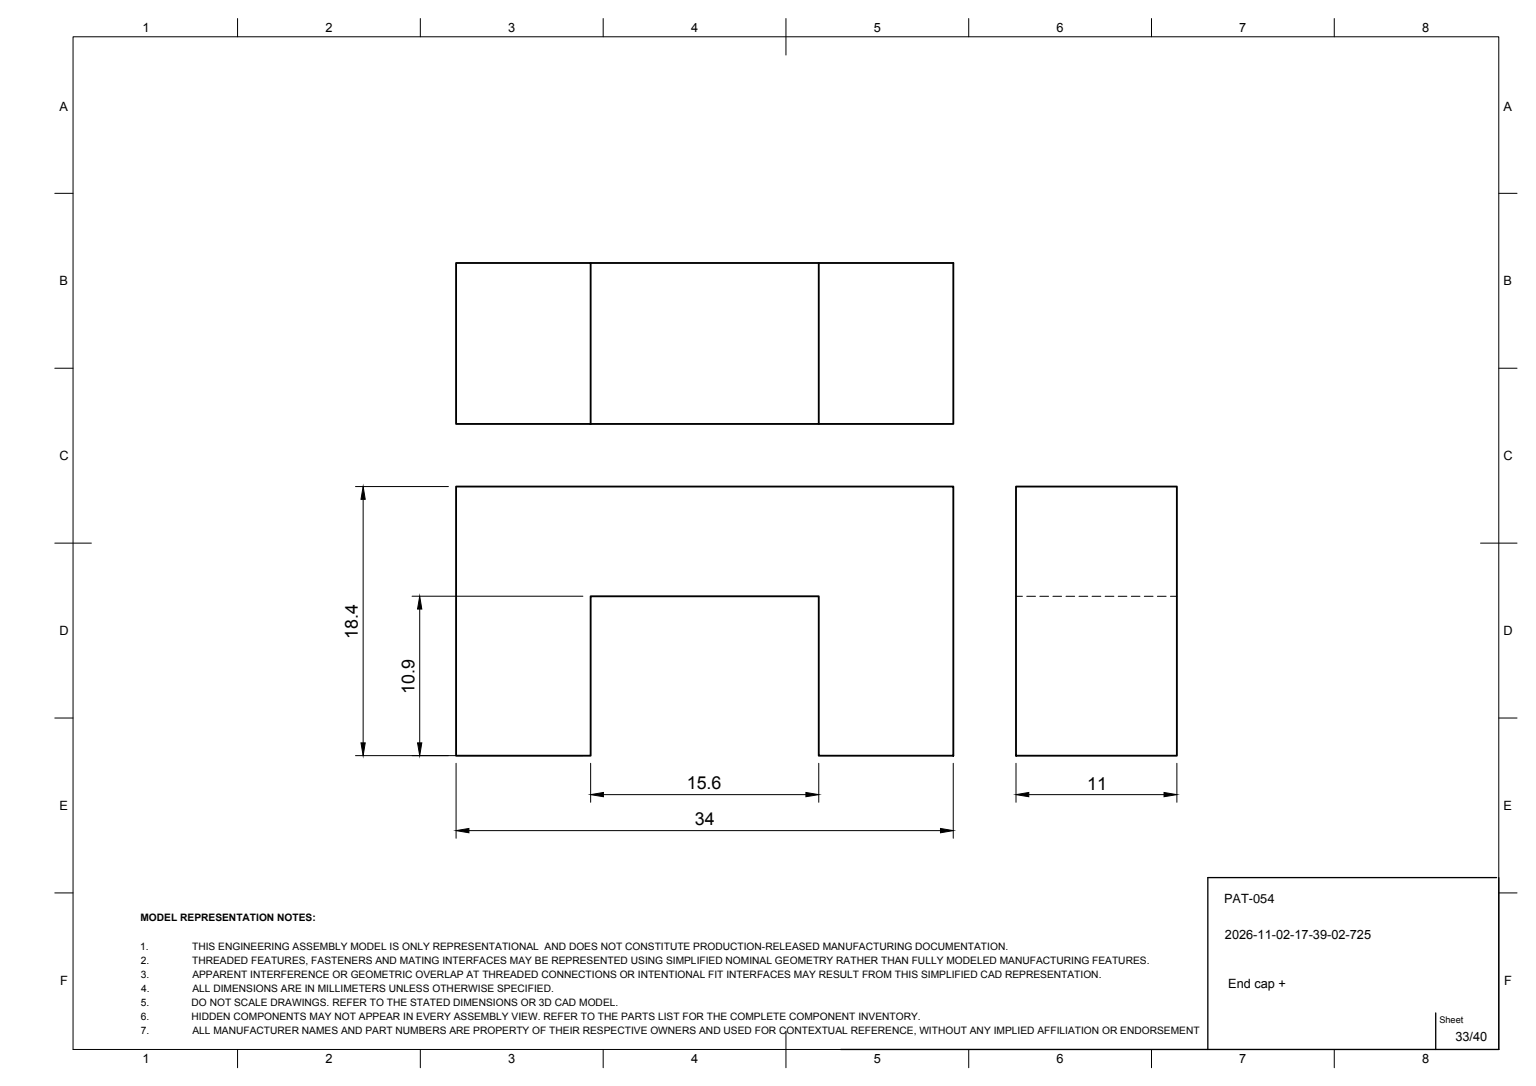
ISO-10303-21;
HEADER;
/* Generated by software containing ST-Developer
 * from STEP Tools, Inc. (www.steptools.com) 
 */

FILE_DESCRIPTION(
/* description */ ('PAT-054'),
/* implementation_level */ '2;1');

FILE_NAME(
/* name */ 'End cap +.step',
/* time_stamp */ '2026-10-29T16:38:13-07:00',
/* author */ (''),
/* organization */ (''),
/* preprocessor_version */ 'ST-DEVELOPER v20.2',
/* originating_system */ 'Autodesk Translation Framework v15.17.0.0',
/* authorisation */ '');

FILE_SCHEMA (('AUTOMOTIVE_DESIGN { 1 0 10303 214 3 1 1 }'));
ENDSEC;

DATA;
#10=MECHANICAL_DESIGN_GEOMETRIC_PRESENTATION_REPRESENTATION('',(#941),#33981);
#838=SHAPE_REPRESENTATION_RELATIONSHIP('SRR','None',#34215,#882);
#882=ADVANCED_BREP_SHAPE_REPRESENTATION('',(#999),#33963);
#941=STYLED_ITEM('',(#34510),#999);
#999=MANIFOLD_SOLID_BREP('Body1',#13053);
#1455=PLANE('',#14365);
#1456=PLANE('',#14366);
#1457=PLANE('',#14367);
#1458=PLANE('',#14368);
#1459=PLANE('',#14369);
#1460=PLANE('',#14370);
#1461=PLANE('',#14371);
#1462=PLANE('',#14372);
#1463=PLANE('',#14373);
#1464=PLANE('',#14374);
#1972=FACE_OUTER_BOUND('',#2872,.T.);
#1973=FACE_OUTER_BOUND('',#2873,.T.);
#1974=FACE_OUTER_BOUND('',#2874,.T.);
#1975=FACE_OUTER_BOUND('',#2875,.T.);
#1976=FACE_OUTER_BOUND('',#2876,.T.);
#1977=FACE_OUTER_BOUND('',#2877,.T.);
#1978=FACE_OUTER_BOUND('',#2878,.T.);
#1979=FACE_OUTER_BOUND('',#2879,.T.);
#1980=FACE_OUTER_BOUND('',#2880,.T.);
#1981=FACE_OUTER_BOUND('',#2881,.T.);
#2872=EDGE_LOOP('',(#10373,#10374,#10375,#10376));
#2873=EDGE_LOOP('',(#10377,#10378,#10379,#10380));
#2874=EDGE_LOOP('',(#10381,#10382,#10383,#10384));
#2875=EDGE_LOOP('',(#10385,#10386,#10387,#10388));
#2876=EDGE_LOOP('',(#10389,#10390,#10391,#10392));
#2877=EDGE_LOOP('',(#10393,#10394,#10395,#10396));
#2878=EDGE_LOOP('',(#10397,#10398,#10399,#10400));
#2879=EDGE_LOOP('',(#10401,#10402,#10403,#10404));
#2880=EDGE_LOOP('',(#10405,#10406,#10407,#10408,#10409,#10410,#10411,#10412));
#2881=EDGE_LOOP('',(#10413,#10414,#10415,#10416,#10417,#10418,#10419,#10420));
#3782=LINE('',#21148,#4716);
#3783=LINE('',#21150,#4717);
#3784=LINE('',#21152,#4718);
#3785=LINE('',#21153,#4719);
#3786=LINE('',#21156,#4720);
#3787=LINE('',#21158,#4721);
#3788=LINE('',#21159,#4722);
#3789=LINE('',#21162,#4723);
#3790=LINE('',#21164,#4724);
#3791=LINE('',#21165,#4725);
#3792=LINE('',#21168,#4726);
#3793=LINE('',#21170,#4727);
#3794=LINE('',#21171,#4728);
#3795=LINE('',#21174,#4729);
#3796=LINE('',#21176,#4730);
#3797=LINE('',#21177,#4731);
#3798=LINE('',#21180,#4732);
#3799=LINE('',#21182,#4733);
#3800=LINE('',#21183,#4734);
#3801=LINE('',#21186,#4735);
#3802=LINE('',#21188,#4736);
#3803=LINE('',#21189,#4737);
#3804=LINE('',#21191,#4738);
#3805=LINE('',#21192,#4739);
#4716=VECTOR('',#17049,1.);
#4717=VECTOR('',#17050,1.);
#4718=VECTOR('',#17051,1.);
#4719=VECTOR('',#17052,1.);
#4720=VECTOR('',#17055,1.);
#4721=VECTOR('',#17056,1.);
#4722=VECTOR('',#17057,1.);
#4723=VECTOR('',#17060,1.);
#4724=VECTOR('',#17061,1.);
#4725=VECTOR('',#17062,1.);
#4726=VECTOR('',#17065,1.);
#4727=VECTOR('',#17066,1.);
#4728=VECTOR('',#17067,1.);
#4729=VECTOR('',#17070,1.);
#4730=VECTOR('',#17071,1.);
#4731=VECTOR('',#17072,1.);
#4732=VECTOR('',#17075,1.);
#4733=VECTOR('',#17076,1.);
#4734=VECTOR('',#17077,1.);
#4735=VECTOR('',#17080,1.);
#4736=VECTOR('',#17081,1.);
#4737=VECTOR('',#17082,1.);
#4738=VECTOR('',#17085,1.);
#4739=VECTOR('',#17086,1.);
#6214=VERTEX_POINT('',#21146);
#6215=VERTEX_POINT('',#21147);
#6216=VERTEX_POINT('',#21149);
#6217=VERTEX_POINT('',#21151);
#6218=VERTEX_POINT('',#21155);
#6219=VERTEX_POINT('',#21157);
#6220=VERTEX_POINT('',#21161);
#6221=VERTEX_POINT('',#21163);
#6222=VERTEX_POINT('',#21167);
#6223=VERTEX_POINT('',#21169);
#6224=VERTEX_POINT('',#21173);
#6225=VERTEX_POINT('',#21175);
#6226=VERTEX_POINT('',#21179);
#6227=VERTEX_POINT('',#21181);
#6228=VERTEX_POINT('',#21185);
#6229=VERTEX_POINT('',#21187);
#7686=EDGE_CURVE('',#6214,#6215,#3782,.T.);
#7687=EDGE_CURVE('',#6215,#6216,#3783,.T.);
#7688=EDGE_CURVE('',#6217,#6216,#3784,.T.);
#7689=EDGE_CURVE('',#6214,#6217,#3785,.T.);
#7690=EDGE_CURVE('',#6218,#6214,#3786,.T.);
#7691=EDGE_CURVE('',#6219,#6217,#3787,.T.);
#7692=EDGE_CURVE('',#6218,#6219,#3788,.T.);
#7693=EDGE_CURVE('',#6220,#6218,#3789,.T.);
#7694=EDGE_CURVE('',#6221,#6219,#3790,.T.);
#7695=EDGE_CURVE('',#6220,#6221,#3791,.T.);
#7696=EDGE_CURVE('',#6222,#6220,#3792,.T.);
#7697=EDGE_CURVE('',#6223,#6221,#3793,.T.);
#7698=EDGE_CURVE('',#6222,#6223,#3794,.T.);
#7699=EDGE_CURVE('',#6224,#6222,#3795,.T.);
#7700=EDGE_CURVE('',#6225,#6223,#3796,.T.);
#7701=EDGE_CURVE('',#6224,#6225,#3797,.T.);
#7702=EDGE_CURVE('',#6226,#6224,#3798,.T.);
#7703=EDGE_CURVE('',#6227,#6225,#3799,.T.);
#7704=EDGE_CURVE('',#6226,#6227,#3800,.T.);
#7705=EDGE_CURVE('',#6228,#6226,#3801,.T.);
#7706=EDGE_CURVE('',#6229,#6227,#3802,.T.);
#7707=EDGE_CURVE('',#6228,#6229,#3803,.T.);
#7708=EDGE_CURVE('',#6215,#6228,#3804,.T.);
#7709=EDGE_CURVE('',#6216,#6229,#3805,.T.);
#10373=ORIENTED_EDGE('',*,*,#7686,.T.);
#10374=ORIENTED_EDGE('',*,*,#7687,.T.);
#10375=ORIENTED_EDGE('',*,*,#7688,.F.);
#10376=ORIENTED_EDGE('',*,*,#7689,.F.);
#10377=ORIENTED_EDGE('',*,*,#7690,.T.);
#10378=ORIENTED_EDGE('',*,*,#7689,.T.);
#10379=ORIENTED_EDGE('',*,*,#7691,.F.);
#10380=ORIENTED_EDGE('',*,*,#7692,.F.);
#10381=ORIENTED_EDGE('',*,*,#7693,.T.);
#10382=ORIENTED_EDGE('',*,*,#7692,.T.);
#10383=ORIENTED_EDGE('',*,*,#7694,.F.);
#10384=ORIENTED_EDGE('',*,*,#7695,.F.);
#10385=ORIENTED_EDGE('',*,*,#7696,.T.);
#10386=ORIENTED_EDGE('',*,*,#7695,.T.);
#10387=ORIENTED_EDGE('',*,*,#7697,.F.);
#10388=ORIENTED_EDGE('',*,*,#7698,.F.);
#10389=ORIENTED_EDGE('',*,*,#7699,.T.);
#10390=ORIENTED_EDGE('',*,*,#7698,.T.);
#10391=ORIENTED_EDGE('',*,*,#7700,.F.);
#10392=ORIENTED_EDGE('',*,*,#7701,.F.);
#10393=ORIENTED_EDGE('',*,*,#7702,.T.);
#10394=ORIENTED_EDGE('',*,*,#7701,.T.);
#10395=ORIENTED_EDGE('',*,*,#7703,.F.);
#10396=ORIENTED_EDGE('',*,*,#7704,.F.);
#10397=ORIENTED_EDGE('',*,*,#7705,.T.);
#10398=ORIENTED_EDGE('',*,*,#7704,.T.);
#10399=ORIENTED_EDGE('',*,*,#7706,.F.);
#10400=ORIENTED_EDGE('',*,*,#7707,.F.);
#10401=ORIENTED_EDGE('',*,*,#7708,.T.);
#10402=ORIENTED_EDGE('',*,*,#7707,.T.);
#10403=ORIENTED_EDGE('',*,*,#7709,.F.);
#10404=ORIENTED_EDGE('',*,*,#7687,.F.);
#10405=ORIENTED_EDGE('',*,*,#7709,.T.);
#10406=ORIENTED_EDGE('',*,*,#7706,.T.);
#10407=ORIENTED_EDGE('',*,*,#7703,.T.);
#10408=ORIENTED_EDGE('',*,*,#7700,.T.);
#10409=ORIENTED_EDGE('',*,*,#7697,.T.);
#10410=ORIENTED_EDGE('',*,*,#7694,.T.);
#10411=ORIENTED_EDGE('',*,*,#7691,.T.);
#10412=ORIENTED_EDGE('',*,*,#7688,.T.);
#10413=ORIENTED_EDGE('',*,*,#7708,.F.);
#10414=ORIENTED_EDGE('',*,*,#7686,.F.);
#10415=ORIENTED_EDGE('',*,*,#7690,.F.);
#10416=ORIENTED_EDGE('',*,*,#7693,.F.);
#10417=ORIENTED_EDGE('',*,*,#7696,.F.);
#10418=ORIENTED_EDGE('',*,*,#7699,.F.);
#10419=ORIENTED_EDGE('',*,*,#7702,.F.);
#10420=ORIENTED_EDGE('',*,*,#7705,.F.);
#12684=ADVANCED_FACE('',(#1972),#1455,.T.);
#12685=ADVANCED_FACE('',(#1973),#1456,.T.);
#12686=ADVANCED_FACE('',(#1974),#1457,.T.);
#12687=ADVANCED_FACE('',(#1975),#1458,.T.);
#12688=ADVANCED_FACE('',(#1976),#1459,.T.);
#12689=ADVANCED_FACE('',(#1977),#1460,.T.);
#12690=ADVANCED_FACE('',(#1978),#1461,.T.);
#12691=ADVANCED_FACE('',(#1979),#1462,.T.);
#12692=ADVANCED_FACE('',(#1980),#1463,.T.);
#12693=ADVANCED_FACE('',(#1981),#1464,.F.);
#13053=CLOSED_SHELL('',(#12684,#12685,#12686,#12687,#12688,#12689,#12690,
#12691,#12692,#12693));
#14364=AXIS2_PLACEMENT_3D('',#21144,#17045,#17046);
#14365=AXIS2_PLACEMENT_3D('',#21145,#17047,#17048);
#14366=AXIS2_PLACEMENT_3D('',#21154,#17053,#17054);
#14367=AXIS2_PLACEMENT_3D('',#21160,#17058,#17059);
#14368=AXIS2_PLACEMENT_3D('',#21166,#17063,#17064);
#14369=AXIS2_PLACEMENT_3D('',#21172,#17068,#17069);
#14370=AXIS2_PLACEMENT_3D('',#21178,#17073,#17074);
#14371=AXIS2_PLACEMENT_3D('',#21184,#17078,#17079);
#14372=AXIS2_PLACEMENT_3D('',#21190,#17083,#17084);
#14373=AXIS2_PLACEMENT_3D('',#21193,#17087,#17088);
#14374=AXIS2_PLACEMENT_3D('',#21194,#17089,#17090);
#17045=DIRECTION('axis',(0.,0.,1.));
#17046=DIRECTION('refdir',(1.,0.,0.));
#17047=DIRECTION('center_axis',(0.,0.,1.));
#17048=DIRECTION('ref_axis',(0.,-1.,0.));
#17049=DIRECTION('',(0.,-1.,0.));
#17050=DIRECTION('',(1.,0.,0.));
#17051=DIRECTION('',(0.,-1.,0.));
#17052=DIRECTION('',(1.,0.,0.));
#17053=DIRECTION('center_axis',(0.,1.,0.));
#17054=DIRECTION('ref_axis',(0.,0.,1.));
#17055=DIRECTION('',(0.,0.,1.));
#17056=DIRECTION('',(0.,0.,1.));
#17057=DIRECTION('',(1.,0.,0.));
#17058=DIRECTION('center_axis',(0.,0.,-1.));
#17059=DIRECTION('ref_axis',(0.,1.,0.));
#17060=DIRECTION('',(0.,1.,0.));
#17061=DIRECTION('',(0.,1.,0.));
#17062=DIRECTION('',(1.,0.,0.));
#17063=DIRECTION('center_axis',(0.,-1.,0.));
#17064=DIRECTION('ref_axis',(0.,0.,-1.));
#17065=DIRECTION('',(0.,0.,-1.));
#17066=DIRECTION('',(0.,0.,-1.));
#17067=DIRECTION('',(1.,0.,0.));
#17068=DIRECTION('center_axis',(0.,0.,-1.));
#17069=DIRECTION('ref_axis',(0.,1.,0.));
#17070=DIRECTION('',(0.,1.,0.));
#17071=DIRECTION('',(0.,1.,0.));
#17072=DIRECTION('',(1.,0.,0.));
#17073=DIRECTION('center_axis',(0.,1.,0.));
#17074=DIRECTION('ref_axis',(0.,0.,1.));
#17075=DIRECTION('',(0.,0.,1.));
#17076=DIRECTION('',(0.,0.,1.));
#17077=DIRECTION('',(1.,0.,0.));
#17078=DIRECTION('center_axis',(0.,0.,-1.));
#17079=DIRECTION('ref_axis',(0.,1.,0.));
#17080=DIRECTION('',(0.,1.,0.));
#17081=DIRECTION('',(0.,1.,0.));
#17082=DIRECTION('',(1.,0.,0.));
#17083=DIRECTION('center_axis',(0.,-1.,0.));
#17084=DIRECTION('ref_axis',(0.,0.,-1.));
#17085=DIRECTION('',(0.,0.,-1.));
#17086=DIRECTION('',(0.,0.,-1.));
#17087=DIRECTION('center_axis',(1.,0.,0.));
#17088=DIRECTION('ref_axis',(0.,0.,-1.));
#17089=DIRECTION('center_axis',(1.,0.,0.));
#17090=DIRECTION('ref_axis',(0.,0.,-1.));
#21144=CARTESIAN_POINT('',(0.,0.,0.));
#21145=CARTESIAN_POINT('Origin',(1.97,1.7,2.3));
#21146=CARTESIAN_POINT('',(1.97,1.7,2.3));
#21147=CARTESIAN_POINT('',(1.97,-1.7,2.3));
#21148=CARTESIAN_POINT('',(1.97,1.7,2.3));
#21149=CARTESIAN_POINT('',(3.07,-1.7,2.3));
#21150=CARTESIAN_POINT('',(1.97,-1.7,2.3));
#21151=CARTESIAN_POINT('',(3.07,1.7,2.3));
#21152=CARTESIAN_POINT('',(3.07,1.7,2.3));
#21153=CARTESIAN_POINT('',(1.97,1.7,2.3));
#21154=CARTESIAN_POINT('Origin',(1.97,1.7,0.46));
#21155=CARTESIAN_POINT('',(1.97,1.7,0.46));
#21156=CARTESIAN_POINT('',(1.97,1.7,0.46));
#21157=CARTESIAN_POINT('',(3.07,1.7,0.46));
#21158=CARTESIAN_POINT('',(3.07,1.7,0.46));
#21159=CARTESIAN_POINT('',(1.97,1.7,0.46));
#21160=CARTESIAN_POINT('Origin',(1.97,0.78,0.46));
#21161=CARTESIAN_POINT('',(1.97,0.78,0.46));
#21162=CARTESIAN_POINT('',(1.97,0.78,0.46));
#21163=CARTESIAN_POINT('',(3.07,0.78,0.46));
#21164=CARTESIAN_POINT('',(3.07,0.78,0.46));
#21165=CARTESIAN_POINT('',(1.97,0.78,0.46));
#21166=CARTESIAN_POINT('Origin',(1.97,0.78,1.55));
#21167=CARTESIAN_POINT('',(1.97,0.78,1.55));
#21168=CARTESIAN_POINT('',(1.97,0.78,1.55));
#21169=CARTESIAN_POINT('',(3.07,0.78,1.55));
#21170=CARTESIAN_POINT('',(3.07,0.78,1.55));
#21171=CARTESIAN_POINT('',(1.97,0.78,1.55));
#21172=CARTESIAN_POINT('Origin',(1.97,-0.78,1.55));
#21173=CARTESIAN_POINT('',(1.97,-0.78,1.55));
#21174=CARTESIAN_POINT('',(1.97,-0.78,1.55));
#21175=CARTESIAN_POINT('',(3.07,-0.78,1.55));
#21176=CARTESIAN_POINT('',(3.07,-0.78,1.55));
#21177=CARTESIAN_POINT('',(1.97,-0.78,1.55));
#21178=CARTESIAN_POINT('Origin',(1.97,-0.78,0.46));
#21179=CARTESIAN_POINT('',(1.97,-0.78,0.46));
#21180=CARTESIAN_POINT('',(1.97,-0.78,0.46));
#21181=CARTESIAN_POINT('',(3.07,-0.78,0.46));
#21182=CARTESIAN_POINT('',(3.07,-0.78,0.46));
#21183=CARTESIAN_POINT('',(1.97,-0.78,0.46));
#21184=CARTESIAN_POINT('Origin',(1.97,-1.7,0.46));
#21185=CARTESIAN_POINT('',(1.97,-1.7,0.46));
#21186=CARTESIAN_POINT('',(1.97,-1.7,0.46));
#21187=CARTESIAN_POINT('',(3.07,-1.7,0.46));
#21188=CARTESIAN_POINT('',(3.07,-1.7,0.46));
#21189=CARTESIAN_POINT('',(1.97,-1.7,0.46));
#21190=CARTESIAN_POINT('Origin',(1.97,-1.7,2.3));
#21191=CARTESIAN_POINT('',(1.97,-1.7,2.3));
#21192=CARTESIAN_POINT('',(3.07,-1.7,2.3));
#21193=CARTESIAN_POINT('Origin',(3.07,0.,1.38));
#21194=CARTESIAN_POINT('Origin',(1.97,0.,1.38));
#33911=UNCERTAINTY_MEASURE_WITH_UNIT(LENGTH_MEASURE(0.001),#33982,
'DISTANCE_ACCURACY_VALUE',
'Maximum model space distance between geometric entities at asserted c
onnectivities');
#33929=UNCERTAINTY_MEASURE_WITH_UNIT(LENGTH_MEASURE(0.001),#33982,
'DISTANCE_ACCURACY_VALUE',
'Maximum model space distance between geometric entities at asserted c
onnectivities');
#33963=(
GEOMETRIC_REPRESENTATION_CONTEXT(3)
GLOBAL_UNCERTAINTY_ASSIGNED_CONTEXT((#33911))
GLOBAL_UNIT_ASSIGNED_CONTEXT((#33982,#33984,#33985))
REPRESENTATION_CONTEXT('','3D')
);
#33981=(
GEOMETRIC_REPRESENTATION_CONTEXT(3)
GLOBAL_UNCERTAINTY_ASSIGNED_CONTEXT((#33929))
GLOBAL_UNIT_ASSIGNED_CONTEXT((#33982,#33984,#33985))
REPRESENTATION_CONTEXT('','3D')
);
#33982=(
LENGTH_UNIT()
NAMED_UNIT(*)
SI_UNIT(.CENTI.,.METRE.)
);
#33984=(
NAMED_UNIT(*)
PLANE_ANGLE_UNIT()
SI_UNIT($,.RADIAN.)
);
#33985=(
NAMED_UNIT(*)
SI_UNIT($,.STERADIAN.)
SOLID_ANGLE_UNIT()
);
#34019=SHAPE_DEFINITION_REPRESENTATION(#34080,#34215);
#34080=PRODUCT_DEFINITION_SHAPE('',$,#34267);
#34215=SHAPE_REPRESENTATION('',(#14364),#33963);
#34233=PRODUCT_DEFINITION_CONTEXT('part definition',#34388,'design');
#34267=PRODUCT_DEFINITION('End cap +','End cap +',#34318,#34233);
#34318=PRODUCT_DEFINITION_FORMATION('',$,#34423);
#34388=APPLICATION_CONTEXT(
'Core Data for Automotive Mechanical Design Process');
#34389=PRODUCT_CONTEXT('part definition',#34388,'mechanical');
#34423=PRODUCT('End cap +','End cap +','End cap +',(#34389));
#34504=COLOUR_RGB('Sky Blue',0.24,0.69,0.87);
#34505=FILL_AREA_STYLE_COLOUR('',#34504);
#34506=FILL_AREA_STYLE('',(#34505));
#34507=SURFACE_STYLE_FILL_AREA(#34506);
#34508=SURFACE_SIDE_STYLE('',(#34507));
#34509=SURFACE_STYLE_USAGE(.BOTH.,#34508);
#34510=PRESENTATION_STYLE_ASSIGNMENT((#34509));
ENDSEC;
END-ISO-10303-21;
